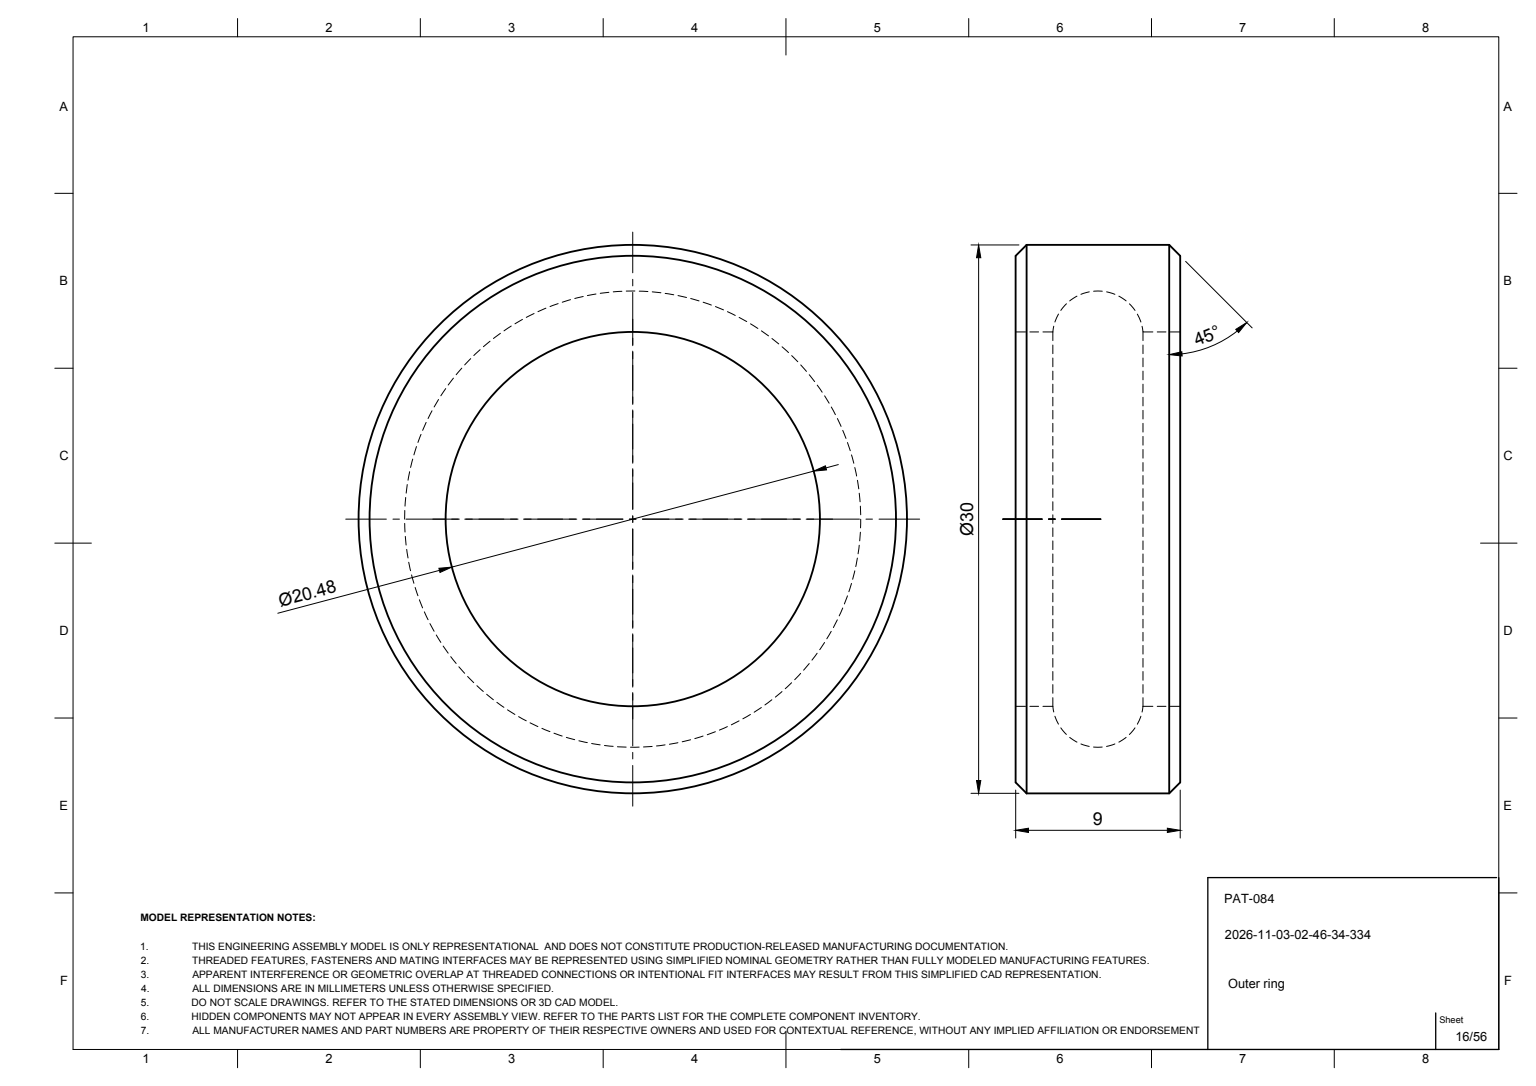
ISO-10303-21;
HEADER;
/* Generated by software containing ST-Developer
 * from STEP Tools, Inc. (www.steptools.com) 
 */

FILE_DESCRIPTION(
/* description */ ('Quick-return (Whitworth) mechanism'),
/* implementation_level */ '2;1');

FILE_NAME(
/* name */ 'Outer ring.step',
/* time_stamp */ '2026-10-28T03:25:57-07:00',
/* author */ (''),
/* organization */ (''),
/* preprocessor_version */ 'ST-DEVELOPER v20.2',
/* originating_system */ 'Autodesk Translation Framework v15.17.0.0',
/* authorisation */ '');

FILE_SCHEMA (('AUTOMOTIVE_DESIGN { 1 0 10303 214 3 1 1 }'));
ENDSEC;

DATA;
#10=MECHANICAL_DESIGN_GEOMETRIC_PRESENTATION_REPRESENTATION('',(#499),#14878);
#351=CONICAL_SURFACE('',#8741,1.47,0.785398163397449);
#352=CONICAL_SURFACE('',#8745,1.47,0.785398163397449);
#365=TOROIDAL_SURFACE('',#8730,1.,0.247676);
#411=SHAPE_REPRESENTATION_RELATIONSHIP('SRR','None',#15080,#455);
#455=ADVANCED_BREP_SHAPE_REPRESENTATION('',(#551),#14837);
#499=STYLED_ITEM('',(#15406),#551);
#551=MANIFOLD_SOLID_BREP('Body1',#7853);
#695=FACE_BOUND('',#1778,.T.);
#696=FACE_BOUND('',#1783,.T.);
#858=PLANE('',#8738);
#859=PLANE('',#8747);
#1205=FACE_OUTER_BOUND('',#1775,.T.);
#1206=FACE_OUTER_BOUND('',#1776,.T.);
#1207=FACE_OUTER_BOUND('',#1777,.T.);
#1208=FACE_OUTER_BOUND('',#1779,.T.);
#1209=FACE_OUTER_BOUND('',#1780,.T.);
#1210=FACE_OUTER_BOUND('',#1781,.T.);
#1211=FACE_OUTER_BOUND('',#1782,.T.);
#1212=FACE_OUTER_BOUND('',#1784,.T.);
#1775=EDGE_LOOP('',(#5950,#5951,#5952,#5953,#5954,#5955));
#1776=EDGE_LOOP('',(#5956,#5957,#5958,#5959,#5960));
#1777=EDGE_LOOP('',(#5961));
#1778=EDGE_LOOP('',(#5962));
#1779=EDGE_LOOP('',(#5963,#5964,#5965,#5966));
#1780=EDGE_LOOP('',(#5967,#5968,#5969,#5970));
#1781=EDGE_LOOP('',(#5971,#5972,#5973,#5974));
#1782=EDGE_LOOP('',(#5975));
#1783=EDGE_LOOP('',(#5976));
#1784=EDGE_LOOP('',(#5977,#5978,#5979,#5980,#5981));
#2331=LINE('',#12840,#2854);
#2332=LINE('',#12849,#2855);
#2333=LINE('',#12853,#2856);
#2334=LINE('',#12857,#2857);
#2335=LINE('',#12860,#2858);
#2854=VECTOR('',#10266,1.023815);
#2855=VECTOR('',#10277,1.47);
#2856=VECTOR('',#10282,1.5);
#2857=VECTOR('',#10287,1.47);
#2858=VECTOR('',#10292,1.023815);
#3391=CIRCLE('',#8731,1.023815);
#3392=CIRCLE('',#8732,1.023815);
#3393=CIRCLE('',#8733,0.247676);
#3394=CIRCLE('',#8734,1.023815);
#3395=CIRCLE('',#8735,1.023815);
#3396=CIRCLE('',#8737,1.023815);
#3397=CIRCLE('',#8739,1.44);
#3398=CIRCLE('',#8740,1.023815);
#3399=CIRCLE('',#8742,1.5);
#3400=CIRCLE('',#8744,1.5);
#3401=CIRCLE('',#8746,1.44);
#3861=VERTEX_POINT('',#12828);
#3862=VERTEX_POINT('',#12829);
#3863=VERTEX_POINT('',#12832);
#3864=VERTEX_POINT('',#12834);
#3865=VERTEX_POINT('',#12838);
#3866=VERTEX_POINT('',#12842);
#3867=VERTEX_POINT('',#12844);
#3868=VERTEX_POINT('',#12847);
#3869=VERTEX_POINT('',#12851);
#3870=VERTEX_POINT('',#12855);
#4632=EDGE_CURVE('',#3861,#3862,#3391,.T.);
#4633=EDGE_CURVE('',#3862,#3861,#3392,.T.);
#4634=EDGE_CURVE('',#3862,#3863,#3393,.T.);
#4635=EDGE_CURVE('',#3864,#3863,#3394,.T.);
#4636=EDGE_CURVE('',#3863,#3864,#3395,.T.);
#4637=EDGE_CURVE('',#3865,#3865,#3396,.T.);
#4638=EDGE_CURVE('',#3865,#3864,#2331,.T.);
#4639=EDGE_CURVE('',#3866,#3866,#3397,.T.);
#4640=EDGE_CURVE('',#3867,#3867,#3398,.T.);
#4641=EDGE_CURVE('',#3868,#3868,#3399,.T.);
#4642=EDGE_CURVE('',#3868,#3866,#2332,.T.);
#4643=EDGE_CURVE('',#3869,#3869,#3400,.T.);
#4644=EDGE_CURVE('',#3869,#3868,#2333,.T.);
#4645=EDGE_CURVE('',#3870,#3870,#3401,.T.);
#4646=EDGE_CURVE('',#3870,#3869,#2334,.T.);
#4647=EDGE_CURVE('',#3861,#3867,#2335,.T.);
#5950=ORIENTED_EDGE('',*,*,#4632,.F.);
#5951=ORIENTED_EDGE('',*,*,#4633,.F.);
#5952=ORIENTED_EDGE('',*,*,#4634,.T.);
#5953=ORIENTED_EDGE('',*,*,#4635,.F.);
#5954=ORIENTED_EDGE('',*,*,#4636,.F.);
#5955=ORIENTED_EDGE('',*,*,#4634,.F.);
#5956=ORIENTED_EDGE('',*,*,#4637,.T.);
#5957=ORIENTED_EDGE('',*,*,#4638,.T.);
#5958=ORIENTED_EDGE('',*,*,#4635,.T.);
#5959=ORIENTED_EDGE('',*,*,#4636,.T.);
#5960=ORIENTED_EDGE('',*,*,#4638,.F.);
#5961=ORIENTED_EDGE('',*,*,#4639,.F.);
#5962=ORIENTED_EDGE('',*,*,#4640,.T.);
#5963=ORIENTED_EDGE('',*,*,#4641,.F.);
#5964=ORIENTED_EDGE('',*,*,#4642,.T.);
#5965=ORIENTED_EDGE('',*,*,#4639,.T.);
#5966=ORIENTED_EDGE('',*,*,#4642,.F.);
#5967=ORIENTED_EDGE('',*,*,#4643,.F.);
#5968=ORIENTED_EDGE('',*,*,#4644,.T.);
#5969=ORIENTED_EDGE('',*,*,#4641,.T.);
#5970=ORIENTED_EDGE('',*,*,#4644,.F.);
#5971=ORIENTED_EDGE('',*,*,#4645,.F.);
#5972=ORIENTED_EDGE('',*,*,#4646,.T.);
#5973=ORIENTED_EDGE('',*,*,#4643,.T.);
#5974=ORIENTED_EDGE('',*,*,#4646,.F.);
#5975=ORIENTED_EDGE('',*,*,#4645,.T.);
#5976=ORIENTED_EDGE('',*,*,#4637,.F.);
#5977=ORIENTED_EDGE('',*,*,#4632,.T.);
#5978=ORIENTED_EDGE('',*,*,#4633,.T.);
#5979=ORIENTED_EDGE('',*,*,#4647,.T.);
#5980=ORIENTED_EDGE('',*,*,#4640,.F.);
#5981=ORIENTED_EDGE('',*,*,#4647,.F.);
#7289=CYLINDRICAL_SURFACE('',#8736,1.023815);
#7290=CYLINDRICAL_SURFACE('',#8743,1.5);
#7291=CYLINDRICAL_SURFACE('',#8748,1.023815);
#7536=ADVANCED_FACE('',(#1205),#365,.F.);
#7537=ADVANCED_FACE('',(#1206),#7289,.F.);
#7538=ADVANCED_FACE('',(#1207,#695),#858,.T.);
#7539=ADVANCED_FACE('',(#1208),#351,.T.);
#7540=ADVANCED_FACE('',(#1209),#7290,.T.);
#7541=ADVANCED_FACE('',(#1210),#352,.T.);
#7542=ADVANCED_FACE('',(#1211,#696),#859,.T.);
#7543=ADVANCED_FACE('',(#1212),#7291,.F.);
#7853=CLOSED_SHELL('',(#7536,#7537,#7538,#7539,#7540,#7541,#7542,#7543));
#8729=AXIS2_PLACEMENT_3D('',#12826,#10248,#10249);
#8730=AXIS2_PLACEMENT_3D('',#12827,#10250,#10251);
#8731=AXIS2_PLACEMENT_3D('',#12830,#10252,#10253);
#8732=AXIS2_PLACEMENT_3D('',#12831,#10254,#10255);
#8733=AXIS2_PLACEMENT_3D('',#12833,#10256,#10257);
#8734=AXIS2_PLACEMENT_3D('',#12835,#10258,#10259);
#8735=AXIS2_PLACEMENT_3D('',#12836,#10260,#10261);
#8736=AXIS2_PLACEMENT_3D('',#12837,#10262,#10263);
#8737=AXIS2_PLACEMENT_3D('',#12839,#10264,#10265);
#8738=AXIS2_PLACEMENT_3D('',#12841,#10267,#10268);
#8739=AXIS2_PLACEMENT_3D('',#12843,#10269,#10270);
#8740=AXIS2_PLACEMENT_3D('',#12845,#10271,#10272);
#8741=AXIS2_PLACEMENT_3D('',#12846,#10273,#10274);
#8742=AXIS2_PLACEMENT_3D('',#12848,#10275,#10276);
#8743=AXIS2_PLACEMENT_3D('',#12850,#10278,#10279);
#8744=AXIS2_PLACEMENT_3D('',#12852,#10280,#10281);
#8745=AXIS2_PLACEMENT_3D('',#12854,#10283,#10284);
#8746=AXIS2_PLACEMENT_3D('',#12856,#10285,#10286);
#8747=AXIS2_PLACEMENT_3D('',#12858,#10288,#10289);
#8748=AXIS2_PLACEMENT_3D('',#12859,#10290,#10291);
#10248=DIRECTION('axis',(0.,0.,1.));
#10249=DIRECTION('refdir',(1.,0.,0.));
#10250=DIRECTION('center_axis',(0.,-1.,0.));
#10251=DIRECTION('ref_axis',(0.,0.,-1.));
#10252=DIRECTION('center_axis',(0.,-1.,0.));
#10253=DIRECTION('ref_axis',(1.,0.,0.));
#10254=DIRECTION('center_axis',(0.,-1.,0.));
#10255=DIRECTION('ref_axis',(1.,0.,0.));
#10256=DIRECTION('center_axis',(1.,0.,1.22464679914735E-16));
#10257=DIRECTION('ref_axis',(-1.22464679914735E-16,0.,1.));
#10258=DIRECTION('center_axis',(0.,1.,0.));
#10259=DIRECTION('ref_axis',(1.,0.,0.));
#10260=DIRECTION('center_axis',(0.,1.,0.));
#10261=DIRECTION('ref_axis',(1.,0.,0.));
#10262=DIRECTION('center_axis',(0.,-1.,0.));
#10263=DIRECTION('ref_axis',(1.,0.,0.));
#10264=DIRECTION('center_axis',(0.,-1.,0.));
#10265=DIRECTION('ref_axis',(1.,0.,0.));
#10266=DIRECTION('',(0.,1.,0.));
#10267=DIRECTION('center_axis',(0.,1.,0.));
#10268=DIRECTION('ref_axis',(0.,0.,1.));
#10269=DIRECTION('center_axis',(0.,-1.,0.));
#10270=DIRECTION('ref_axis',(1.,0.,0.));
#10271=DIRECTION('center_axis',(0.,-1.,0.));
#10272=DIRECTION('ref_axis',(1.,0.,0.));
#10273=DIRECTION('center_axis',(0.,-1.,0.));
#10274=DIRECTION('ref_axis',(1.,0.,0.));
#10275=DIRECTION('center_axis',(0.,-1.,0.));
#10276=DIRECTION('ref_axis',(1.,0.,0.));
#10277=DIRECTION('',(0.707106781186548,0.707106781186547,8.65956056235494E-17));
#10278=DIRECTION('center_axis',(0.,-1.,0.));
#10279=DIRECTION('ref_axis',(1.,0.,0.));
#10280=DIRECTION('center_axis',(0.,-1.,0.));
#10281=DIRECTION('ref_axis',(1.,0.,0.));
#10282=DIRECTION('',(0.,1.,0.));
#10283=DIRECTION('center_axis',(0.,1.,0.));
#10284=DIRECTION('ref_axis',(1.,0.,0.));
#10285=DIRECTION('center_axis',(0.,-1.,0.));
#10286=DIRECTION('ref_axis',(1.,0.,0.));
#10287=DIRECTION('',(-0.707106781186548,0.707106781186547,-8.65956056235494E-17));
#10288=DIRECTION('center_axis',(0.,-1.,0.));
#10289=DIRECTION('ref_axis',(0.,0.,-1.));
#10290=DIRECTION('center_axis',(0.,-1.,0.));
#10291=DIRECTION('ref_axis',(1.,0.,0.));
#10292=DIRECTION('',(0.,1.,0.));
#12826=CARTESIAN_POINT('',(0.,0.,0.));
#12827=CARTESIAN_POINT('Origin',(0.,0.,0.));
#12828=CARTESIAN_POINT('',(-1.023815,0.246528389340863,-1.25381176266905E-16));
#12829=CARTESIAN_POINT('',(-1.25381176266905E-16,0.246528389340863,1.023815));
#12830=CARTESIAN_POINT('Origin',(0.,0.246528389340863,0.));
#12831=CARTESIAN_POINT('Origin',(0.,0.246528389340863,0.));
#12832=CARTESIAN_POINT('',(-1.25381176266905E-16,-0.246528389340863,1.023815));
#12833=CARTESIAN_POINT('Origin',(-1.22464679914735E-16,0.,1.));
#12834=CARTESIAN_POINT('',(-1.023815,-0.246528389340863,1.25381176266905E-16));
#12835=CARTESIAN_POINT('Origin',(0.,-0.246528389340863,0.));
#12836=CARTESIAN_POINT('Origin',(0.,-0.246528389340863,0.));
#12837=CARTESIAN_POINT('Origin',(0.,0.,0.));
#12838=CARTESIAN_POINT('',(-1.023815,-0.45,-1.25381176266905E-16));
#12839=CARTESIAN_POINT('Origin',(0.,-0.45,0.));
#12840=CARTESIAN_POINT('',(-1.023815,0.,-1.25381176266905E-16));
#12841=CARTESIAN_POINT('Origin',(1.44,0.45,0.));
#12842=CARTESIAN_POINT('',(-1.44,0.45,-1.76349139077219E-16));
#12843=CARTESIAN_POINT('Origin',(0.,0.45,0.));
#12844=CARTESIAN_POINT('',(-1.023815,0.45,-1.25381176266905E-16));
#12845=CARTESIAN_POINT('Origin',(0.,0.45,0.));
#12846=CARTESIAN_POINT('Origin',(0.,0.42,0.));
#12847=CARTESIAN_POINT('',(-1.5,0.39,-1.83697019872103E-16));
#12848=CARTESIAN_POINT('Origin',(0.,0.39,0.));
#12849=CARTESIAN_POINT('',(-1.47,0.42,-1.80023079474661E-16));
#12850=CARTESIAN_POINT('Origin',(0.,0.,0.));
#12851=CARTESIAN_POINT('',(-1.5,-0.39,-1.83697019872103E-16));
#12852=CARTESIAN_POINT('Origin',(0.,-0.39,0.));
#12853=CARTESIAN_POINT('',(-1.5,0.,-1.83697019872103E-16));
#12854=CARTESIAN_POINT('Origin',(0.,-0.42,0.));
#12855=CARTESIAN_POINT('',(-1.44,-0.45,-1.76349139077219E-16));
#12856=CARTESIAN_POINT('Origin',(0.,-0.45,0.));
#12857=CARTESIAN_POINT('',(-1.47,-0.42,-1.80023079474661E-16));
#12858=CARTESIAN_POINT('Origin',(1.023815,-0.45,0.));
#12859=CARTESIAN_POINT('Origin',(0.,0.,0.));
#12860=CARTESIAN_POINT('',(-1.023815,0.,-1.25381176266905E-16));
#14783=UNCERTAINTY_MEASURE_WITH_UNIT(LENGTH_MEASURE(0.001),#14879,
'DISTANCE_ACCURACY_VALUE',
'Maximum model space distance between geometric entities at asserted c
onnectivities');
#14824=UNCERTAINTY_MEASURE_WITH_UNIT(LENGTH_MEASURE(0.001),#14879,
'DISTANCE_ACCURACY_VALUE',
'Maximum model space distance between geometric entities at asserted c
onnectivities');
#14837=(
GEOMETRIC_REPRESENTATION_CONTEXT(3)
GLOBAL_UNCERTAINTY_ASSIGNED_CONTEXT((#14783))
GLOBAL_UNIT_ASSIGNED_CONTEXT((#14879,#14881,#14882))
REPRESENTATION_CONTEXT('','3D')
);
#14878=(
GEOMETRIC_REPRESENTATION_CONTEXT(3)
GLOBAL_UNCERTAINTY_ASSIGNED_CONTEXT((#14824))
GLOBAL_UNIT_ASSIGNED_CONTEXT((#14879,#14881,#14882))
REPRESENTATION_CONTEXT('','3D')
);
#14879=(
LENGTH_UNIT()
NAMED_UNIT(*)
SI_UNIT(.CENTI.,.METRE.)
);
#14881=(
NAMED_UNIT(*)
PLANE_ANGLE_UNIT()
SI_UNIT($,.RADIAN.)
);
#14882=(
NAMED_UNIT(*)
SI_UNIT($,.STERADIAN.)
SOLID_ANGLE_UNIT()
);
#14895=SHAPE_DEFINITION_REPRESENTATION(#14948,#15080);
#14948=PRODUCT_DEFINITION_SHAPE('',$,#15134);
#15080=SHAPE_REPRESENTATION('',(#8729),#14837);
#15121=PRODUCT_DEFINITION_CONTEXT('part definition',#15282,'design');
#15134=PRODUCT_DEFINITION('Outer ring','Outer ring',#15187,#15121);
#15187=PRODUCT_DEFINITION_FORMATION('',$,#15296);
#15282=APPLICATION_CONTEXT(
'Core Data for Automotive Mechanical Design Process');
#15283=PRODUCT_CONTEXT('part definition',#15282,'mechanical');
#15296=PRODUCT('Outer ring','Outer ring','Outer ring',(#15283));
#15400=COLOUR_RGB('Grey',0.48,0.52,0.57);
#15401=FILL_AREA_STYLE_COLOUR('',#15400);
#15402=FILL_AREA_STYLE('',(#15401));
#15403=SURFACE_STYLE_FILL_AREA(#15402);
#15404=SURFACE_SIDE_STYLE('',(#15403));
#15405=SURFACE_STYLE_USAGE(.BOTH.,#15404);
#15406=PRESENTATION_STYLE_ASSIGNMENT((#15405));
ENDSEC;
END-ISO-10303-21;
